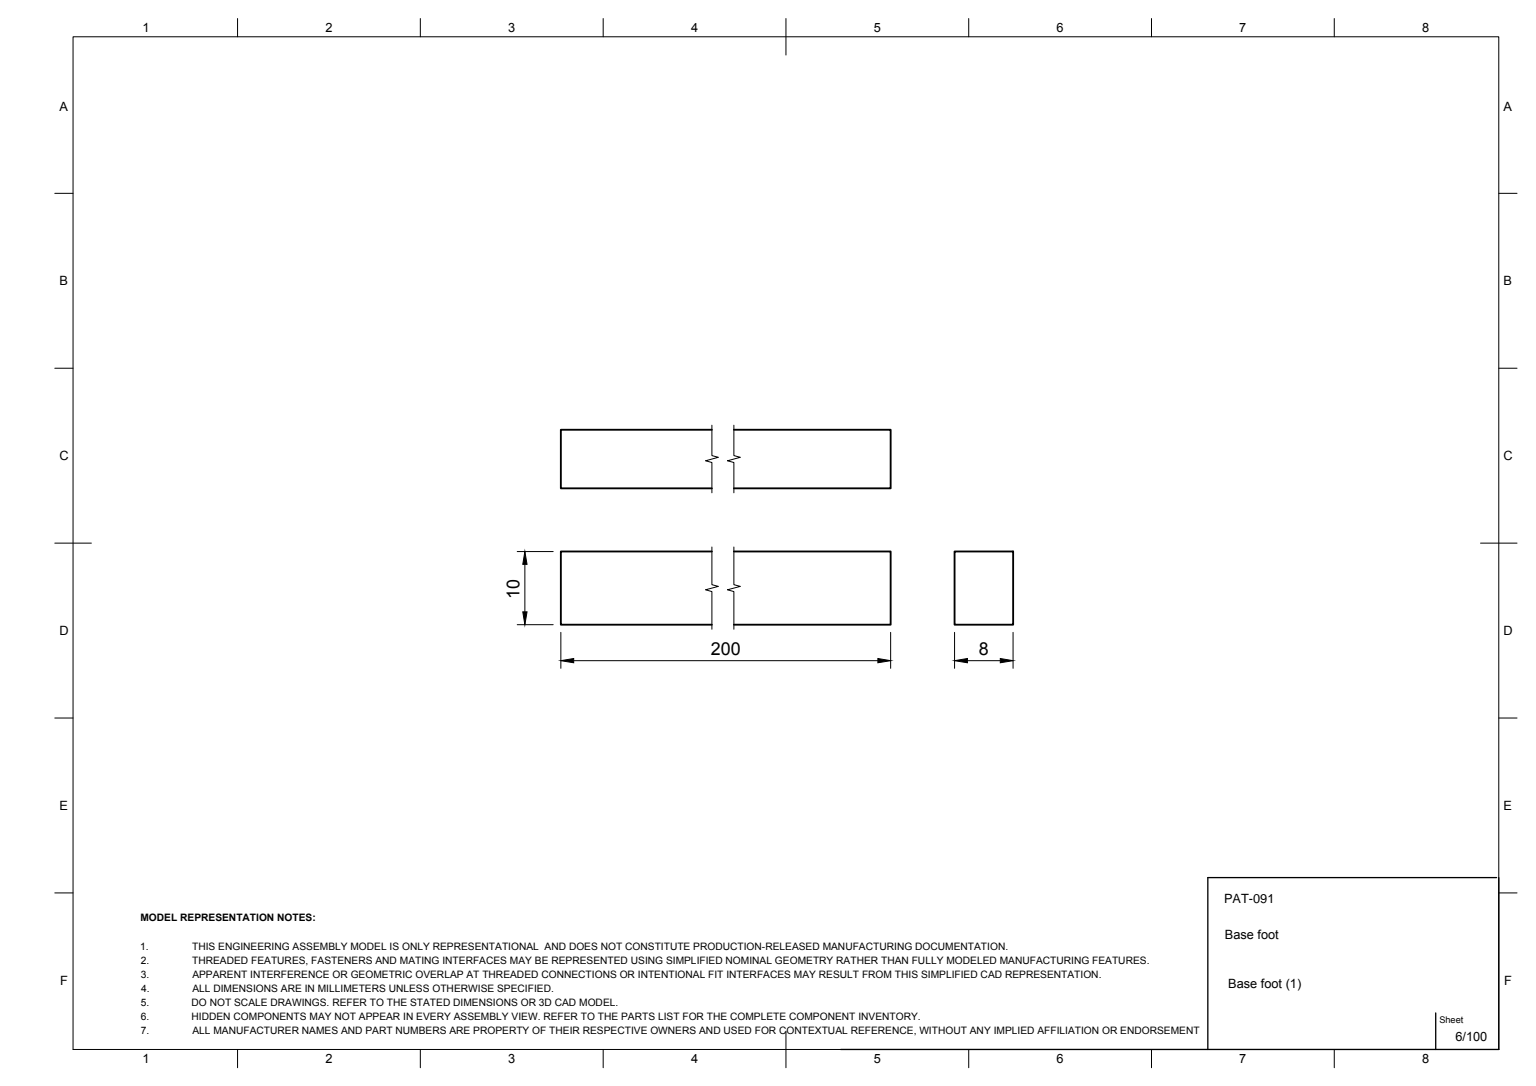
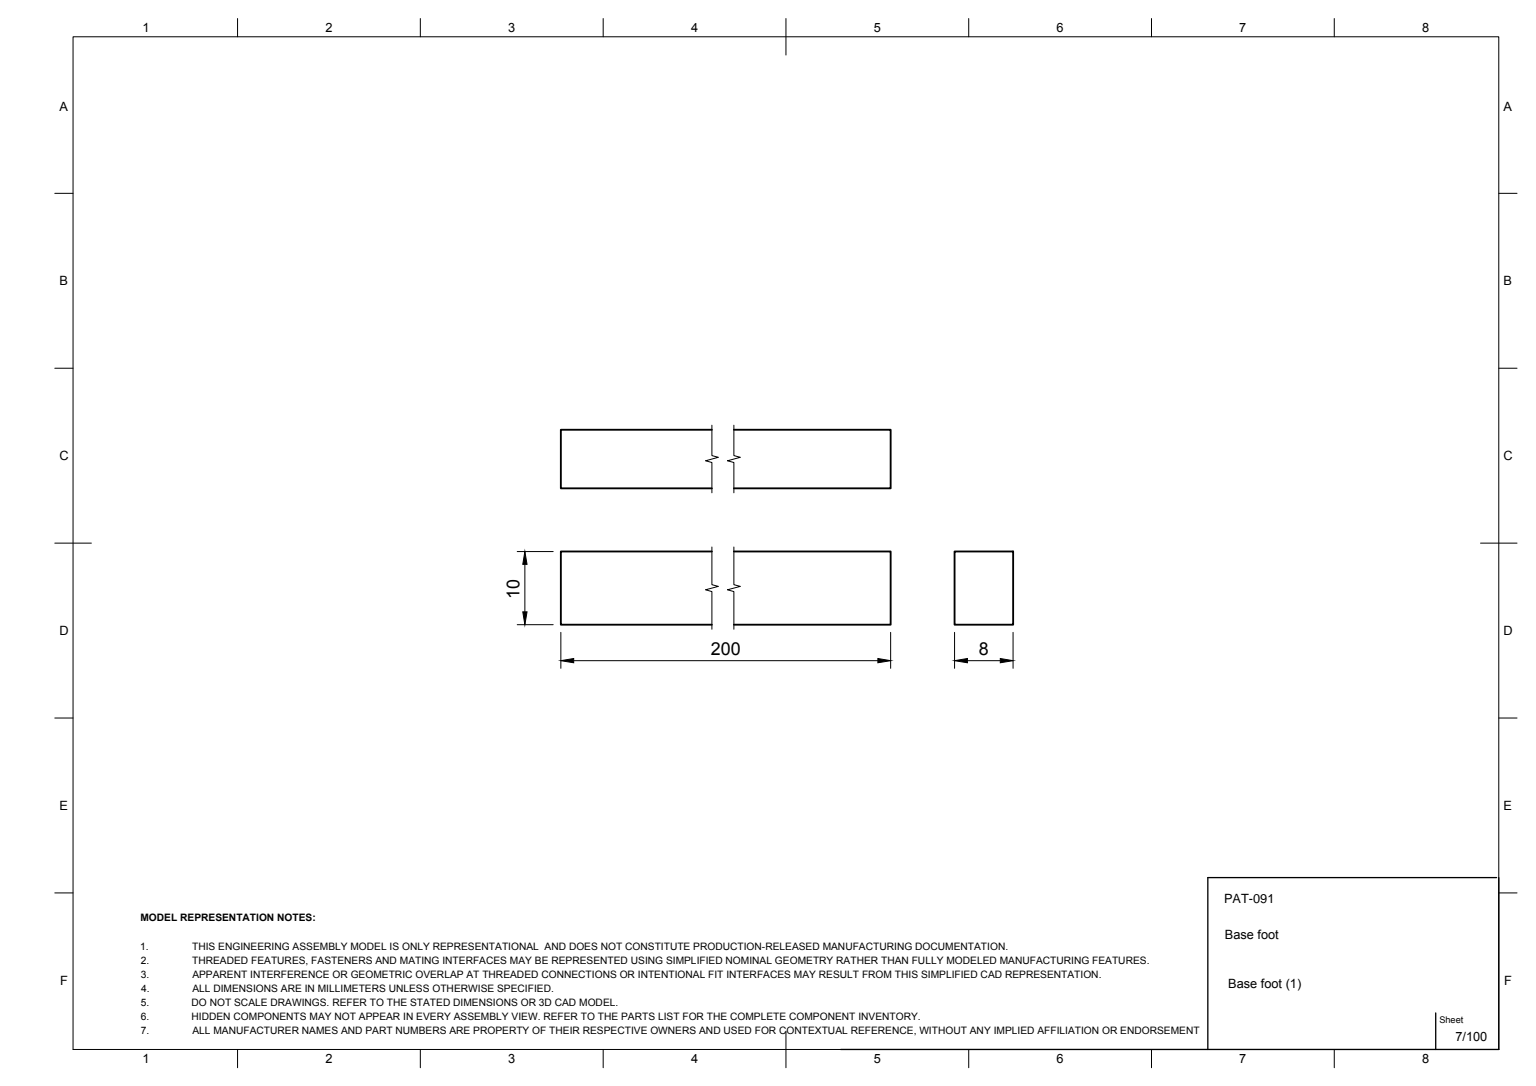
ISO-10303-21;
HEADER;
/* Generated by software containing ST-Developer
 * from STEP Tools, Inc. (www.steptools.com) 
 */

FILE_DESCRIPTION(
/* description */ ('PAT-091'),
/* implementation_level */ '2;1');

FILE_NAME(
/* name */ 'Base foot.step',
/* time_stamp */ '2026-10-27T15:34:44-07:00',
/* author */ (''),
/* organization */ (''),
/* preprocessor_version */ 'ST-DEVELOPER v20.2',
/* originating_system */ 'Autodesk Translation Framework v15.17.0.0',
/* authorisation */ '');

FILE_SCHEMA (('AUTOMOTIVE_DESIGN { 1 0 10303 214 3 1 1 }'));
ENDSEC;

DATA;
#10=MECHANICAL_DESIGN_GEOMETRIC_PRESENTATION_REPRESENTATION('',(#972),#25100);
#752=SHAPE_REPRESENTATION_RELATIONSHIP('SRR','None',#25513,#862);
#862=ADVANCED_BREP_SHAPE_REPRESENTATION('',(#1096),#24983);
#972=STYLED_ITEM('',(#26170),#1096);
#1096=MANIFOLD_SOLID_BREP('Body1',#13249);
#1646=PLANE('',#14619);
#1647=PLANE('',#14620);
#1648=PLANE('',#14621);
#1649=PLANE('',#14622);
#1650=PLANE('',#14623);
#1651=PLANE('',#14624);
#2077=FACE_OUTER_BOUND('',#2911,.T.);
#2078=FACE_OUTER_BOUND('',#2912,.T.);
#2079=FACE_OUTER_BOUND('',#2913,.T.);
#2080=FACE_OUTER_BOUND('',#2914,.T.);
#2081=FACE_OUTER_BOUND('',#2915,.T.);
#2082=FACE_OUTER_BOUND('',#2916,.T.);
#2911=EDGE_LOOP('',(#9044,#9045,#9046,#9047));
#2912=EDGE_LOOP('',(#9048,#9049,#9050,#9051));
#2913=EDGE_LOOP('',(#9052,#9053,#9054,#9055));
#2914=EDGE_LOOP('',(#9056,#9057,#9058,#9059));
#2915=EDGE_LOOP('',(#9060,#9061,#9062,#9063));
#2916=EDGE_LOOP('',(#9064,#9065,#9066,#9067));
#4144=LINE('',#21055,#4884);
#4145=LINE('',#21057,#4885);
#4146=LINE('',#21059,#4886);
#4147=LINE('',#21060,#4887);
#4148=LINE('',#21063,#4888);
#4149=LINE('',#21065,#4889);
#4150=LINE('',#21066,#4890);
#4151=LINE('',#21069,#4891);
#4152=LINE('',#21071,#4892);
#4153=LINE('',#21072,#4893);
#4154=LINE('',#21074,#4894);
#4155=LINE('',#21075,#4895);
#4884=VECTOR('',#16558,1.);
#4885=VECTOR('',#16559,1.);
#4886=VECTOR('',#16560,1.);
#4887=VECTOR('',#16561,1.);
#4888=VECTOR('',#16564,1.);
#4889=VECTOR('',#16565,1.);
#4890=VECTOR('',#16566,1.);
#4891=VECTOR('',#16569,1.);
#4892=VECTOR('',#16570,1.);
#4893=VECTOR('',#16571,1.);
#4894=VECTOR('',#16574,1.);
#4895=VECTOR('',#16575,1.);
#6407=VERTEX_POINT('',#21053);
#6408=VERTEX_POINT('',#21054);
#6409=VERTEX_POINT('',#21056);
#6410=VERTEX_POINT('',#21058);
#6411=VERTEX_POINT('',#21062);
#6412=VERTEX_POINT('',#21064);
#6413=VERTEX_POINT('',#21068);
#6414=VERTEX_POINT('',#21070);
#7457=EDGE_CURVE('',#6407,#6408,#4144,.T.);
#7458=EDGE_CURVE('',#6408,#6409,#4145,.T.);
#7459=EDGE_CURVE('',#6410,#6409,#4146,.T.);
#7460=EDGE_CURVE('',#6407,#6410,#4147,.T.);
#7461=EDGE_CURVE('',#6411,#6407,#4148,.T.);
#7462=EDGE_CURVE('',#6412,#6410,#4149,.T.);
#7463=EDGE_CURVE('',#6411,#6412,#4150,.T.);
#7464=EDGE_CURVE('',#6413,#6411,#4151,.T.);
#7465=EDGE_CURVE('',#6414,#6412,#4152,.T.);
#7466=EDGE_CURVE('',#6413,#6414,#4153,.T.);
#7467=EDGE_CURVE('',#6408,#6413,#4154,.T.);
#7468=EDGE_CURVE('',#6409,#6414,#4155,.T.);
#9044=ORIENTED_EDGE('',*,*,#7457,.T.);
#9045=ORIENTED_EDGE('',*,*,#7458,.T.);
#9046=ORIENTED_EDGE('',*,*,#7459,.F.);
#9047=ORIENTED_EDGE('',*,*,#7460,.F.);
#9048=ORIENTED_EDGE('',*,*,#7461,.T.);
#9049=ORIENTED_EDGE('',*,*,#7460,.T.);
#9050=ORIENTED_EDGE('',*,*,#7462,.F.);
#9051=ORIENTED_EDGE('',*,*,#7463,.F.);
#9052=ORIENTED_EDGE('',*,*,#7464,.T.);
#9053=ORIENTED_EDGE('',*,*,#7463,.T.);
#9054=ORIENTED_EDGE('',*,*,#7465,.F.);
#9055=ORIENTED_EDGE('',*,*,#7466,.F.);
#9056=ORIENTED_EDGE('',*,*,#7467,.T.);
#9057=ORIENTED_EDGE('',*,*,#7466,.T.);
#9058=ORIENTED_EDGE('',*,*,#7468,.F.);
#9059=ORIENTED_EDGE('',*,*,#7458,.F.);
#9060=ORIENTED_EDGE('',*,*,#7468,.T.);
#9061=ORIENTED_EDGE('',*,*,#7465,.T.);
#9062=ORIENTED_EDGE('',*,*,#7462,.T.);
#9063=ORIENTED_EDGE('',*,*,#7459,.T.);
#9064=ORIENTED_EDGE('',*,*,#7467,.F.);
#9065=ORIENTED_EDGE('',*,*,#7457,.F.);
#9066=ORIENTED_EDGE('',*,*,#7461,.F.);
#9067=ORIENTED_EDGE('',*,*,#7464,.F.);
#12444=ADVANCED_FACE('',(#2077),#1646,.T.);
#12445=ADVANCED_FACE('',(#2078),#1647,.T.);
#12446=ADVANCED_FACE('',(#2079),#1648,.T.);
#12447=ADVANCED_FACE('',(#2080),#1649,.T.);
#12448=ADVANCED_FACE('',(#2081),#1650,.T.);
#12449=ADVANCED_FACE('',(#2082),#1651,.F.);
#13249=CLOSED_SHELL('',(#12444,#12445,#12446,#12447,#12448,#12449));
#14618=AXIS2_PLACEMENT_3D('',#21051,#16554,#16555);
#14619=AXIS2_PLACEMENT_3D('',#21052,#16556,#16557);
#14620=AXIS2_PLACEMENT_3D('',#21061,#16562,#16563);
#14621=AXIS2_PLACEMENT_3D('',#21067,#16567,#16568);
#14622=AXIS2_PLACEMENT_3D('',#21073,#16572,#16573);
#14623=AXIS2_PLACEMENT_3D('',#21076,#16576,#16577);
#14624=AXIS2_PLACEMENT_3D('',#21077,#16578,#16579);
#16554=DIRECTION('axis',(0.,0.,1.));
#16555=DIRECTION('refdir',(1.,0.,0.));
#16556=DIRECTION('center_axis',(0.,1.,0.));
#16557=DIRECTION('ref_axis',(-1.,0.,0.));
#16558=DIRECTION('',(-1.,0.,0.));
#16559=DIRECTION('',(0.,0.,1.));
#16560=DIRECTION('',(-1.,0.,0.));
#16561=DIRECTION('',(0.,0.,1.));
#16562=DIRECTION('center_axis',(1.,0.,0.));
#16563=DIRECTION('ref_axis',(0.,1.,0.));
#16564=DIRECTION('',(0.,1.,0.));
#16565=DIRECTION('',(0.,1.,0.));
#16566=DIRECTION('',(0.,0.,1.));
#16567=DIRECTION('center_axis',(0.,-1.,0.));
#16568=DIRECTION('ref_axis',(1.,0.,0.));
#16569=DIRECTION('',(1.,0.,0.));
#16570=DIRECTION('',(1.,0.,0.));
#16571=DIRECTION('',(0.,0.,1.));
#16572=DIRECTION('center_axis',(-1.,0.,0.));
#16573=DIRECTION('ref_axis',(0.,-1.,0.));
#16574=DIRECTION('',(0.,-1.,0.));
#16575=DIRECTION('',(0.,-1.,0.));
#16576=DIRECTION('center_axis',(0.,0.,1.));
#16577=DIRECTION('ref_axis',(1.,0.,0.));
#16578=DIRECTION('center_axis',(0.,0.,1.));
#16579=DIRECTION('ref_axis',(1.,0.,0.));
#21051=CARTESIAN_POINT('',(0.,0.,0.));
#21052=CARTESIAN_POINT('Origin',(-2.,10.,-0.8));
#21053=CARTESIAN_POINT('',(-2.,10.,-1.8));
#21054=CARTESIAN_POINT('',(-3.,10.,-1.8));
#21055=CARTESIAN_POINT('',(-2.25,10.,-1.8));
#21056=CARTESIAN_POINT('',(-3.,10.,0.));
#21057=CARTESIAN_POINT('',(-3.,10.,-0.8));
#21058=CARTESIAN_POINT('',(-2.,10.,0.));
#21059=CARTESIAN_POINT('',(-2.,10.,0.));
#21060=CARTESIAN_POINT('',(-2.,10.,-0.8));
#21061=CARTESIAN_POINT('Origin',(-2.,-10.,-0.8));
#21062=CARTESIAN_POINT('',(-2.,-10.,-1.8));
#21063=CARTESIAN_POINT('',(-2.,-5.,-1.8));
#21064=CARTESIAN_POINT('',(-2.,-10.,0.));
#21065=CARTESIAN_POINT('',(-2.,-10.,0.));
#21066=CARTESIAN_POINT('',(-2.,-10.,-0.8));
#21067=CARTESIAN_POINT('Origin',(-3.,-10.,-0.8));
#21068=CARTESIAN_POINT('',(-3.,-10.,-1.8));
#21069=CARTESIAN_POINT('',(-2.75,-10.,-1.8));
#21070=CARTESIAN_POINT('',(-3.,-10.,0.));
#21071=CARTESIAN_POINT('',(-3.,-10.,0.));
#21072=CARTESIAN_POINT('',(-3.,-10.,-0.8));
#21073=CARTESIAN_POINT('Origin',(-3.,10.,-0.8));
#21074=CARTESIAN_POINT('',(-3.,5.,-1.8));
#21075=CARTESIAN_POINT('',(-3.,10.,0.));
#21076=CARTESIAN_POINT('Origin',(-2.5,0.,0.));
#21077=CARTESIAN_POINT('Origin',(-2.5,0.,-1.8));
#24862=UNCERTAINTY_MEASURE_WITH_UNIT(LENGTH_MEASURE(0.001),#25101,
'DISTANCE_ACCURACY_VALUE',
'Maximum model space distance between geometric entities at asserted c
onnectivities');
#24979=UNCERTAINTY_MEASURE_WITH_UNIT(LENGTH_MEASURE(0.001),#25101,
'DISTANCE_ACCURACY_VALUE',
'Maximum model space distance between geometric entities at asserted c
onnectivities');
#24983=(
GEOMETRIC_REPRESENTATION_CONTEXT(3)
GLOBAL_UNCERTAINTY_ASSIGNED_CONTEXT((#24862))
GLOBAL_UNIT_ASSIGNED_CONTEXT((#25101,#25103,#25104))
REPRESENTATION_CONTEXT('','3D')
);
#25100=(
GEOMETRIC_REPRESENTATION_CONTEXT(3)
GLOBAL_UNCERTAINTY_ASSIGNED_CONTEXT((#24979))
GLOBAL_UNIT_ASSIGNED_CONTEXT((#25101,#25103,#25104))
REPRESENTATION_CONTEXT('','3D')
);
#25101=(
LENGTH_UNIT()
NAMED_UNIT(*)
SI_UNIT(.CENTI.,.METRE.)
);
#25103=(
NAMED_UNIT(*)
PLANE_ANGLE_UNIT()
SI_UNIT($,.RADIAN.)
);
#25104=(
NAMED_UNIT(*)
SI_UNIT($,.STERADIAN.)
SOLID_ANGLE_UNIT()
);
#25108=SHAPE_DEFINITION_REPRESENTATION(#25228,#25513);
#25228=PRODUCT_DEFINITION_SHAPE('',$,#25634);
#25513=SHAPE_REPRESENTATION('',(#14618),#24983);
#25630=PRODUCT_DEFINITION_CONTEXT('part definition',#25992,'design');
#25634=PRODUCT_DEFINITION('Base foot','Base foot',#25754,#25630);
#25754=PRODUCT_DEFINITION_FORMATION('',$,#25997);
#25992=APPLICATION_CONTEXT(
'Core Data for Automotive Mechanical Design Process');
#25993=PRODUCT_CONTEXT('part definition',#25992,'mechanical');
#25997=PRODUCT('Base foot','Base foot','Base foot',(#25993));
#26164=COLOUR_RGB('Dark Blue',0.08,0.2,0.34);
#26165=FILL_AREA_STYLE_COLOUR('',#26164);
#26166=FILL_AREA_STYLE('',(#26165));
#26167=SURFACE_STYLE_FILL_AREA(#26166);
#26168=SURFACE_SIDE_STYLE('',(#26167));
#26169=SURFACE_STYLE_USAGE(.BOTH.,#26168);
#26170=PRESENTATION_STYLE_ASSIGNMENT((#26169));
ENDSEC;
END-ISO-10303-21;
